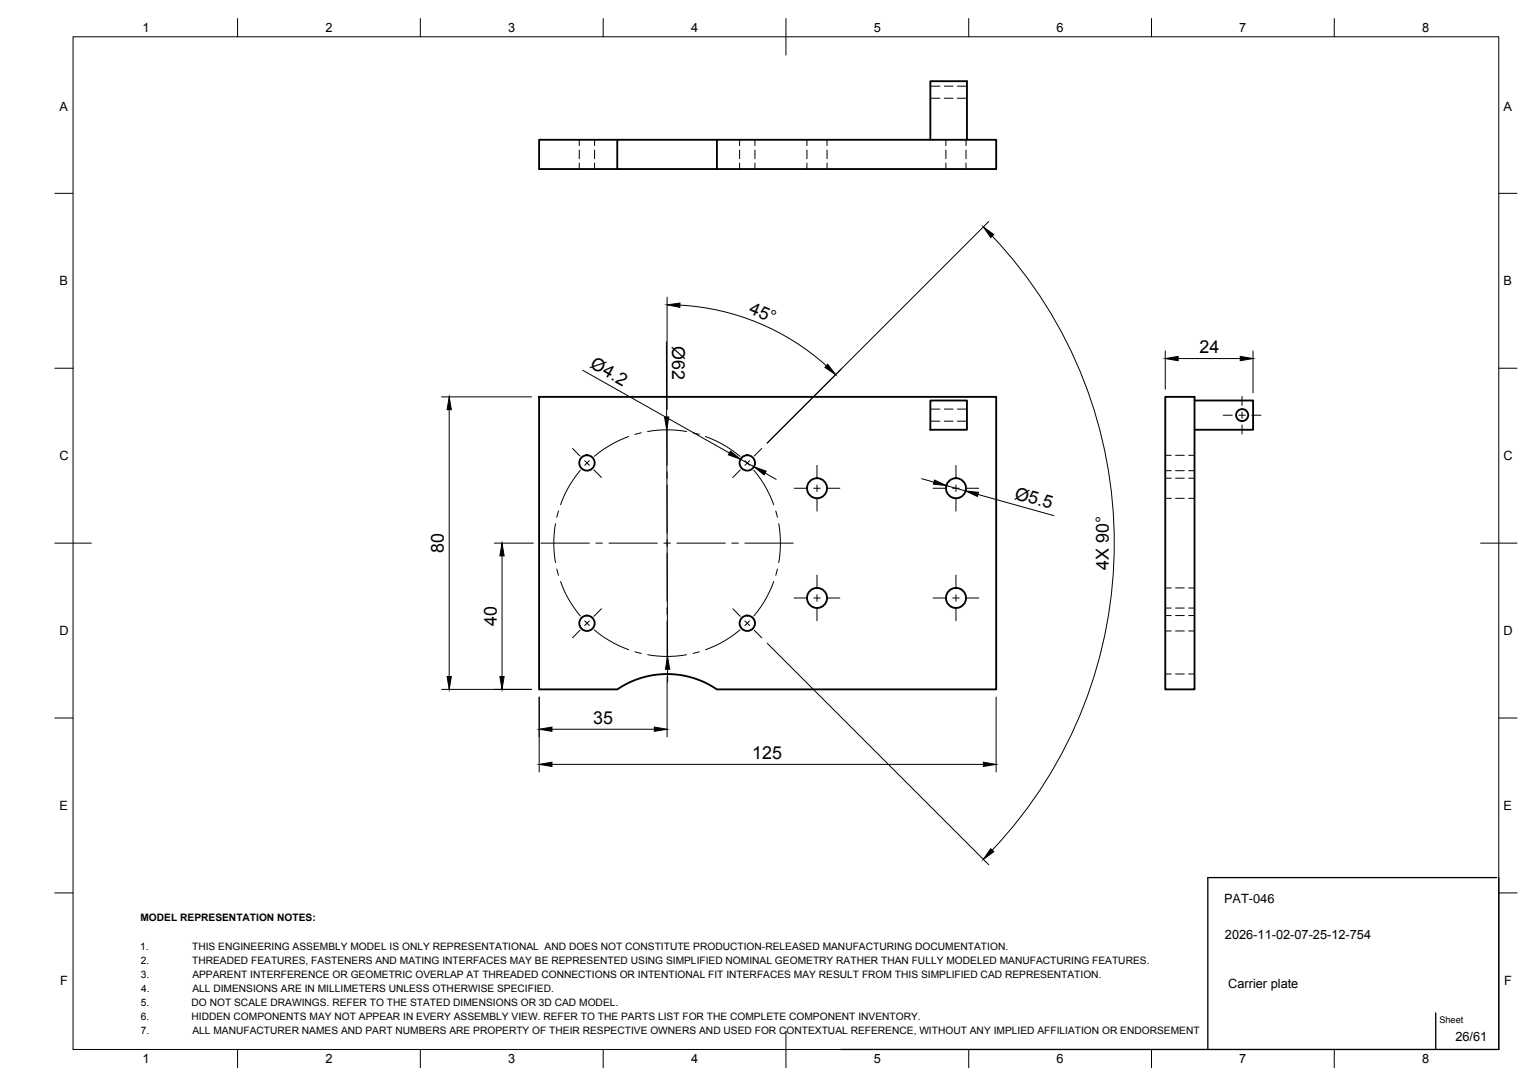
ISO-10303-21;
HEADER;
/* Generated by software containing ST-Developer
 * from STEP Tools, Inc. (www.steptools.com) 
 */

FILE_DESCRIPTION(
/* description */ ('Gear mesh backlash fixture'),
/* implementation_level */ '2;1');

FILE_NAME(
/* name */ 'Carrier plate.step',
/* time_stamp */ '2026-10-28T03:26:00-07:00',
/* author */ (''),
/* organization */ (''),
/* preprocessor_version */ 'ST-DEVELOPER v20.2',
/* originating_system */ 'Autodesk Translation Framework v15.17.0.0',
/* authorisation */ '');

FILE_SCHEMA (('AUTOMOTIVE_DESIGN { 1 0 10303 214 3 1 1 }'));
ENDSEC;

DATA;
#10=MECHANICAL_DESIGN_GEOMETRIC_PRESENTATION_REPRESENTATION('',(#1041),#57900);
#934=SHAPE_REPRESENTATION_RELATIONSHIP('SRR','None',#58131,#984);
#984=ADVANCED_BREP_SHAPE_REPRESENTATION('',(#1105),#57864);
#1041=STYLED_ITEM('',(#58451),#1105);
#1105=MANIFOLD_SOLID_BREP('Body1',#13602);
#1227=FACE_BOUND('',#2760,.T.);
#1228=FACE_BOUND('',#2763,.T.);
#1229=FACE_BOUND('',#2772,.T.);
#1230=FACE_BOUND('',#2773,.T.);
#1231=FACE_BOUND('',#2774,.T.);
#1232=FACE_BOUND('',#2775,.T.);
#1233=FACE_BOUND('',#2776,.T.);
#1234=FACE_BOUND('',#2777,.T.);
#1235=FACE_BOUND('',#2778,.T.);
#1236=FACE_BOUND('',#2779,.T.);
#1237=FACE_BOUND('',#2786,.T.);
#1238=FACE_BOUND('',#2787,.T.);
#1239=FACE_BOUND('',#2788,.T.);
#1240=FACE_BOUND('',#2789,.T.);
#1241=FACE_BOUND('',#2790,.T.);
#1242=FACE_BOUND('',#2791,.T.);
#1243=FACE_BOUND('',#2792,.T.);
#1244=FACE_BOUND('',#2793,.T.);
#1245=FACE_BOUND('',#2794,.T.);
#1440=PLANE('',#14667);
#1441=PLANE('',#14668);
#1442=PLANE('',#14669);
#1443=PLANE('',#14670);
#1444=PLANE('',#14671);
#1445=PLANE('',#14687);
#1446=PLANE('',#14688);
#1447=PLANE('',#14689);
#1448=PLANE('',#14690);
#1449=PLANE('',#14691);
#1450=PLANE('',#14692);
#1451=PLANE('',#14693);
#1905=FACE_OUTER_BOUND('',#2754,.T.);
#1906=FACE_OUTER_BOUND('',#2755,.T.);
#1907=FACE_OUTER_BOUND('',#2756,.T.);
#1908=FACE_OUTER_BOUND('',#2757,.T.);
#1909=FACE_OUTER_BOUND('',#2758,.T.);
#1910=FACE_OUTER_BOUND('',#2759,.T.);
#1911=FACE_OUTER_BOUND('',#2761,.T.);
#1912=FACE_OUTER_BOUND('',#2762,.T.);
#1913=FACE_OUTER_BOUND('',#2764,.T.);
#1914=FACE_OUTER_BOUND('',#2765,.T.);
#1915=FACE_OUTER_BOUND('',#2766,.T.);
#1916=FACE_OUTER_BOUND('',#2767,.T.);
#1917=FACE_OUTER_BOUND('',#2768,.T.);
#1918=FACE_OUTER_BOUND('',#2769,.T.);
#1919=FACE_OUTER_BOUND('',#2770,.T.);
#1920=FACE_OUTER_BOUND('',#2771,.T.);
#1921=FACE_OUTER_BOUND('',#2780,.T.);
#1922=FACE_OUTER_BOUND('',#2781,.T.);
#1923=FACE_OUTER_BOUND('',#2782,.T.);
#1924=FACE_OUTER_BOUND('',#2783,.T.);
#1925=FACE_OUTER_BOUND('',#2784,.T.);
#1926=FACE_OUTER_BOUND('',#2785,.T.);
#2754=EDGE_LOOP('',(#9809,#9810,#9811,#9812));
#2755=EDGE_LOOP('',(#9813,#9814,#9815,#9816));
#2756=EDGE_LOOP('',(#9817,#9818,#9819,#9820));
#2757=EDGE_LOOP('',(#9821,#9822,#9823,#9824));
#2758=EDGE_LOOP('',(#9825,#9826,#9827,#9828));
#2759=EDGE_LOOP('',(#9829,#9830,#9831,#9832));
#2760=EDGE_LOOP('',(#9833));
#2761=EDGE_LOOP('',(#9834,#9835,#9836,#9837));
#2762=EDGE_LOOP('',(#9838,#9839,#9840,#9841));
#2763=EDGE_LOOP('',(#9842));
#2764=EDGE_LOOP('',(#9843,#9844,#9845,#9846));
#2765=EDGE_LOOP('',(#9847,#9848,#9849,#9850));
#2766=EDGE_LOOP('',(#9851,#9852,#9853,#9854));
#2767=EDGE_LOOP('',(#9855,#9856,#9857,#9858));
#2768=EDGE_LOOP('',(#9859,#9860,#9861,#9862));
#2769=EDGE_LOOP('',(#9863,#9864,#9865,#9866));
#2770=EDGE_LOOP('',(#9867,#9868,#9869,#9870));
#2771=EDGE_LOOP('',(#9871,#9872,#9873,#9874,#9875,#9876));
#2772=EDGE_LOOP('',(#9877));
#2773=EDGE_LOOP('',(#9878));
#2774=EDGE_LOOP('',(#9879));
#2775=EDGE_LOOP('',(#9880));
#2776=EDGE_LOOP('',(#9881));
#2777=EDGE_LOOP('',(#9882));
#2778=EDGE_LOOP('',(#9883));
#2779=EDGE_LOOP('',(#9884));
#2780=EDGE_LOOP('',(#9885,#9886,#9887,#9888));
#2781=EDGE_LOOP('',(#9889,#9890,#9891,#9892));
#2782=EDGE_LOOP('',(#9893,#9894,#9895,#9896));
#2783=EDGE_LOOP('',(#9897,#9898,#9899,#9900));
#2784=EDGE_LOOP('',(#9901,#9902,#9903,#9904));
#2785=EDGE_LOOP('',(#9905,#9906,#9907,#9908,#9909,#9910));
#2786=EDGE_LOOP('',(#9911));
#2787=EDGE_LOOP('',(#9912));
#2788=EDGE_LOOP('',(#9913));
#2789=EDGE_LOOP('',(#9914));
#2790=EDGE_LOOP('',(#9915,#9916,#9917,#9918));
#2791=EDGE_LOOP('',(#9919));
#2792=EDGE_LOOP('',(#9920));
#2793=EDGE_LOOP('',(#9921));
#2794=EDGE_LOOP('',(#9922));
#3637=LINE('',#20642,#4526);
#3638=LINE('',#20648,#4527);
#3639=LINE('',#20654,#4528);
#3640=LINE('',#20660,#4529);
#3641=LINE('',#20666,#4530);
#3642=LINE('',#20671,#4531);
#3643=LINE('',#20673,#4532);
#3644=LINE('',#20675,#4533);
#3645=LINE('',#20676,#4534);
#3646=LINE('',#20679,#4535);
#3647=LINE('',#20681,#4536);
#3648=LINE('',#20682,#4537);
#3649=LINE('',#20685,#4538);
#3650=LINE('',#20687,#4539);
#3651=LINE('',#20688,#4540);
#3652=LINE('',#20690,#4541);
#3653=LINE('',#20691,#4542);
#3654=LINE('',#20697,#4543);
#3655=LINE('',#20703,#4544);
#3656=LINE('',#20709,#4545);
#3657=LINE('',#20715,#4546);
#3658=LINE('',#20720,#4547);
#3659=LINE('',#20724,#4548);
#3660=LINE('',#20728,#4549);
#3661=LINE('',#20730,#4550);
#3662=LINE('',#20732,#4551);
#3663=LINE('',#20734,#4552);
#3664=LINE('',#20735,#4553);
#3665=LINE('',#20738,#4554);
#3666=LINE('',#20739,#4555);
#3667=LINE('',#20742,#4556);
#3668=LINE('',#20743,#4557);
#3669=LINE('',#20746,#4558);
#3670=LINE('',#20747,#4559);
#3671=LINE('',#20750,#4560);
#3672=LINE('',#20751,#4561);
#3673=LINE('',#20753,#4562);
#4526=VECTOR('',#16722,0.21);
#4527=VECTOR('',#16729,0.21);
#4528=VECTOR('',#16736,0.210000000000001);
#4529=VECTOR('',#16743,0.210000000000001);
#4530=VECTOR('',#16750,0.164999999999999);
#4531=VECTOR('',#16755,1.);
#4532=VECTOR('',#16756,1.);
#4533=VECTOR('',#16757,1.);
#4534=VECTOR('',#16758,1.);
#4535=VECTOR('',#16761,1.);
#4536=VECTOR('',#16762,1.);
#4537=VECTOR('',#16763,1.);
#4538=VECTOR('',#16766,1.);
#4539=VECTOR('',#16767,1.);
#4540=VECTOR('',#16768,1.);
#4541=VECTOR('',#16771,1.);
#4542=VECTOR('',#16772,1.);
#4543=VECTOR('',#16779,0.275);
#4544=VECTOR('',#16786,0.275);
#4545=VECTOR('',#16793,0.275);
#4546=VECTOR('',#16800,0.275);
#4547=VECTOR('',#16805,1.);
#4548=VECTOR('',#16808,1.);
#4549=VECTOR('',#16813,1.);
#4550=VECTOR('',#16814,1.);
#4551=VECTOR('',#16815,1.);
#4552=VECTOR('',#16816,1.);
#4553=VECTOR('',#16817,1.);
#4554=VECTOR('',#16820,1.);
#4555=VECTOR('',#16821,1.);
#4556=VECTOR('',#16824,1.);
#4557=VECTOR('',#16825,1.);
#4558=VECTOR('',#16828,1.);
#4559=VECTOR('',#16829,1.);
#4560=VECTOR('',#16832,1.);
#4561=VECTOR('',#16833,1.);
#4562=VECTOR('',#16836,1.);
#5407=CIRCLE('',#14653,0.21);
#5408=CIRCLE('',#14654,0.21);
#5409=CIRCLE('',#14656,0.21);
#5410=CIRCLE('',#14657,0.21);
#5411=CIRCLE('',#14659,0.210000000000001);
#5412=CIRCLE('',#14660,0.210000000000001);
#5413=CIRCLE('',#14662,0.210000000000001);
#5414=CIRCLE('',#14663,0.210000000000001);
#5415=CIRCLE('',#14665,0.164999999999999);
#5416=CIRCLE('',#14666,0.164999999999999);
#5417=CIRCLE('',#14673,0.275);
#5418=CIRCLE('',#14674,0.275);
#5419=CIRCLE('',#14676,0.275);
#5420=CIRCLE('',#14677,0.275);
#5421=CIRCLE('',#14679,0.275);
#5422=CIRCLE('',#14680,0.275);
#5423=CIRCLE('',#14682,0.275);
#5424=CIRCLE('',#14683,0.275);
#5425=CIRCLE('',#14685,2.42);
#5426=CIRCLE('',#14686,2.42);
#6093=VERTEX_POINT('',#20639);
#6094=VERTEX_POINT('',#20641);
#6095=VERTEX_POINT('',#20645);
#6096=VERTEX_POINT('',#20647);
#6097=VERTEX_POINT('',#20651);
#6098=VERTEX_POINT('',#20653);
#6099=VERTEX_POINT('',#20657);
#6100=VERTEX_POINT('',#20659);
#6101=VERTEX_POINT('',#20663);
#6102=VERTEX_POINT('',#20665);
#6103=VERTEX_POINT('',#20669);
#6104=VERTEX_POINT('',#20670);
#6105=VERTEX_POINT('',#20672);
#6106=VERTEX_POINT('',#20674);
#6107=VERTEX_POINT('',#20678);
#6108=VERTEX_POINT('',#20680);
#6109=VERTEX_POINT('',#20684);
#6110=VERTEX_POINT('',#20686);
#6111=VERTEX_POINT('',#20694);
#6112=VERTEX_POINT('',#20696);
#6113=VERTEX_POINT('',#20700);
#6114=VERTEX_POINT('',#20702);
#6115=VERTEX_POINT('',#20706);
#6116=VERTEX_POINT('',#20708);
#6117=VERTEX_POINT('',#20712);
#6118=VERTEX_POINT('',#20714);
#6119=VERTEX_POINT('',#20718);
#6120=VERTEX_POINT('',#20719);
#6121=VERTEX_POINT('',#20721);
#6122=VERTEX_POINT('',#20723);
#6123=VERTEX_POINT('',#20727);
#6124=VERTEX_POINT('',#20729);
#6125=VERTEX_POINT('',#20731);
#6126=VERTEX_POINT('',#20733);
#6127=VERTEX_POINT('',#20737);
#6128=VERTEX_POINT('',#20741);
#6129=VERTEX_POINT('',#20745);
#6130=VERTEX_POINT('',#20749);
#7491=EDGE_CURVE('',#6093,#6093,#5407,.T.);
#7492=EDGE_CURVE('',#6093,#6094,#3637,.T.);
#7493=EDGE_CURVE('',#6094,#6094,#5408,.T.);
#7494=EDGE_CURVE('',#6095,#6095,#5409,.T.);
#7495=EDGE_CURVE('',#6095,#6096,#3638,.T.);
#7496=EDGE_CURVE('',#6096,#6096,#5410,.T.);
#7497=EDGE_CURVE('',#6097,#6097,#5411,.T.);
#7498=EDGE_CURVE('',#6097,#6098,#3639,.T.);
#7499=EDGE_CURVE('',#6098,#6098,#5412,.T.);
#7500=EDGE_CURVE('',#6099,#6099,#5413,.T.);
#7501=EDGE_CURVE('',#6099,#6100,#3640,.T.);
#7502=EDGE_CURVE('',#6100,#6100,#5414,.T.);
#7503=EDGE_CURVE('',#6101,#6101,#5415,.T.);
#7504=EDGE_CURVE('',#6101,#6102,#3641,.T.);
#7505=EDGE_CURVE('',#6102,#6102,#5416,.T.);
#7506=EDGE_CURVE('',#6103,#6104,#3642,.T.);
#7507=EDGE_CURVE('',#6104,#6105,#3643,.T.);
#7508=EDGE_CURVE('',#6106,#6105,#3644,.T.);
#7509=EDGE_CURVE('',#6103,#6106,#3645,.T.);
#7510=EDGE_CURVE('',#6107,#6103,#3646,.T.);
#7511=EDGE_CURVE('',#6108,#6106,#3647,.T.);
#7512=EDGE_CURVE('',#6107,#6108,#3648,.T.);
#7513=EDGE_CURVE('',#6109,#6107,#3649,.T.);
#7514=EDGE_CURVE('',#6110,#6108,#3650,.T.);
#7515=EDGE_CURVE('',#6109,#6110,#3651,.T.);
#7516=EDGE_CURVE('',#6104,#6109,#3652,.T.);
#7517=EDGE_CURVE('',#6105,#6110,#3653,.T.);
#7518=EDGE_CURVE('',#6111,#6111,#5417,.T.);
#7519=EDGE_CURVE('',#6111,#6112,#3654,.T.);
#7520=EDGE_CURVE('',#6112,#6112,#5418,.T.);
#7521=EDGE_CURVE('',#6113,#6113,#5419,.T.);
#7522=EDGE_CURVE('',#6113,#6114,#3655,.T.);
#7523=EDGE_CURVE('',#6114,#6114,#5420,.T.);
#7524=EDGE_CURVE('',#6115,#6115,#5421,.T.);
#7525=EDGE_CURVE('',#6115,#6116,#3656,.T.);
#7526=EDGE_CURVE('',#6116,#6116,#5422,.T.);
#7527=EDGE_CURVE('',#6117,#6117,#5423,.T.);
#7528=EDGE_CURVE('',#6117,#6118,#3657,.T.);
#7529=EDGE_CURVE('',#6118,#6118,#5424,.T.);
#7530=EDGE_CURVE('',#6119,#6120,#3658,.T.);
#7531=EDGE_CURVE('',#6121,#6119,#5425,.T.);
#7532=EDGE_CURVE('',#6122,#6121,#3659,.T.);
#7533=EDGE_CURVE('',#6120,#6122,#5426,.T.);
#7534=EDGE_CURVE('',#6119,#6123,#3660,.T.);
#7535=EDGE_CURVE('',#6123,#6124,#3661,.T.);
#7536=EDGE_CURVE('',#6124,#6125,#3662,.T.);
#7537=EDGE_CURVE('',#6125,#6126,#3663,.T.);
#7538=EDGE_CURVE('',#6126,#6121,#3664,.T.);
#7539=EDGE_CURVE('',#6120,#6127,#3665,.T.);
#7540=EDGE_CURVE('',#6127,#6123,#3666,.T.);
#7541=EDGE_CURVE('',#6128,#6126,#3667,.T.);
#7542=EDGE_CURVE('',#6128,#6122,#3668,.T.);
#7543=EDGE_CURVE('',#6129,#6128,#3669,.T.);
#7544=EDGE_CURVE('',#6129,#6125,#3670,.T.);
#7545=EDGE_CURVE('',#6130,#6129,#3671,.T.);
#7546=EDGE_CURVE('',#6130,#6124,#3672,.T.);
#7547=EDGE_CURVE('',#6127,#6130,#3673,.T.);
#9809=ORIENTED_EDGE('',*,*,#7491,.F.);
#9810=ORIENTED_EDGE('',*,*,#7492,.T.);
#9811=ORIENTED_EDGE('',*,*,#7493,.F.);
#9812=ORIENTED_EDGE('',*,*,#7492,.F.);
#9813=ORIENTED_EDGE('',*,*,#7494,.F.);
#9814=ORIENTED_EDGE('',*,*,#7495,.T.);
#9815=ORIENTED_EDGE('',*,*,#7496,.F.);
#9816=ORIENTED_EDGE('',*,*,#7495,.F.);
#9817=ORIENTED_EDGE('',*,*,#7497,.F.);
#9818=ORIENTED_EDGE('',*,*,#7498,.T.);
#9819=ORIENTED_EDGE('',*,*,#7499,.F.);
#9820=ORIENTED_EDGE('',*,*,#7498,.F.);
#9821=ORIENTED_EDGE('',*,*,#7500,.F.);
#9822=ORIENTED_EDGE('',*,*,#7501,.T.);
#9823=ORIENTED_EDGE('',*,*,#7502,.F.);
#9824=ORIENTED_EDGE('',*,*,#7501,.F.);
#9825=ORIENTED_EDGE('',*,*,#7503,.F.);
#9826=ORIENTED_EDGE('',*,*,#7504,.T.);
#9827=ORIENTED_EDGE('',*,*,#7505,.F.);
#9828=ORIENTED_EDGE('',*,*,#7504,.F.);
#9829=ORIENTED_EDGE('',*,*,#7506,.T.);
#9830=ORIENTED_EDGE('',*,*,#7507,.T.);
#9831=ORIENTED_EDGE('',*,*,#7508,.F.);
#9832=ORIENTED_EDGE('',*,*,#7509,.F.);
#9833=ORIENTED_EDGE('',*,*,#7505,.T.);
#9834=ORIENTED_EDGE('',*,*,#7510,.T.);
#9835=ORIENTED_EDGE('',*,*,#7509,.T.);
#9836=ORIENTED_EDGE('',*,*,#7511,.F.);
#9837=ORIENTED_EDGE('',*,*,#7512,.F.);
#9838=ORIENTED_EDGE('',*,*,#7513,.T.);
#9839=ORIENTED_EDGE('',*,*,#7512,.T.);
#9840=ORIENTED_EDGE('',*,*,#7514,.F.);
#9841=ORIENTED_EDGE('',*,*,#7515,.F.);
#9842=ORIENTED_EDGE('',*,*,#7503,.T.);
#9843=ORIENTED_EDGE('',*,*,#7516,.T.);
#9844=ORIENTED_EDGE('',*,*,#7515,.T.);
#9845=ORIENTED_EDGE('',*,*,#7517,.F.);
#9846=ORIENTED_EDGE('',*,*,#7507,.F.);
#9847=ORIENTED_EDGE('',*,*,#7516,.F.);
#9848=ORIENTED_EDGE('',*,*,#7506,.F.);
#9849=ORIENTED_EDGE('',*,*,#7510,.F.);
#9850=ORIENTED_EDGE('',*,*,#7513,.F.);
#9851=ORIENTED_EDGE('',*,*,#7518,.F.);
#9852=ORIENTED_EDGE('',*,*,#7519,.T.);
#9853=ORIENTED_EDGE('',*,*,#7520,.F.);
#9854=ORIENTED_EDGE('',*,*,#7519,.F.);
#9855=ORIENTED_EDGE('',*,*,#7521,.F.);
#9856=ORIENTED_EDGE('',*,*,#7522,.T.);
#9857=ORIENTED_EDGE('',*,*,#7523,.F.);
#9858=ORIENTED_EDGE('',*,*,#7522,.F.);
#9859=ORIENTED_EDGE('',*,*,#7524,.F.);
#9860=ORIENTED_EDGE('',*,*,#7525,.T.);
#9861=ORIENTED_EDGE('',*,*,#7526,.F.);
#9862=ORIENTED_EDGE('',*,*,#7525,.F.);
#9863=ORIENTED_EDGE('',*,*,#7527,.F.);
#9864=ORIENTED_EDGE('',*,*,#7528,.T.);
#9865=ORIENTED_EDGE('',*,*,#7529,.F.);
#9866=ORIENTED_EDGE('',*,*,#7528,.F.);
#9867=ORIENTED_EDGE('',*,*,#7530,.F.);
#9868=ORIENTED_EDGE('',*,*,#7531,.F.);
#9869=ORIENTED_EDGE('',*,*,#7532,.F.);
#9870=ORIENTED_EDGE('',*,*,#7533,.F.);
#9871=ORIENTED_EDGE('',*,*,#7531,.T.);
#9872=ORIENTED_EDGE('',*,*,#7534,.T.);
#9873=ORIENTED_EDGE('',*,*,#7535,.T.);
#9874=ORIENTED_EDGE('',*,*,#7536,.T.);
#9875=ORIENTED_EDGE('',*,*,#7537,.T.);
#9876=ORIENTED_EDGE('',*,*,#7538,.T.);
#9877=ORIENTED_EDGE('',*,*,#7529,.T.);
#9878=ORIENTED_EDGE('',*,*,#7526,.T.);
#9879=ORIENTED_EDGE('',*,*,#7523,.T.);
#9880=ORIENTED_EDGE('',*,*,#7520,.T.);
#9881=ORIENTED_EDGE('',*,*,#7502,.T.);
#9882=ORIENTED_EDGE('',*,*,#7499,.T.);
#9883=ORIENTED_EDGE('',*,*,#7496,.T.);
#9884=ORIENTED_EDGE('',*,*,#7493,.T.);
#9885=ORIENTED_EDGE('',*,*,#7530,.T.);
#9886=ORIENTED_EDGE('',*,*,#7539,.T.);
#9887=ORIENTED_EDGE('',*,*,#7540,.T.);
#9888=ORIENTED_EDGE('',*,*,#7534,.F.);
#9889=ORIENTED_EDGE('',*,*,#7532,.T.);
#9890=ORIENTED_EDGE('',*,*,#7538,.F.);
#9891=ORIENTED_EDGE('',*,*,#7541,.F.);
#9892=ORIENTED_EDGE('',*,*,#7542,.T.);
#9893=ORIENTED_EDGE('',*,*,#7543,.T.);
#9894=ORIENTED_EDGE('',*,*,#7541,.T.);
#9895=ORIENTED_EDGE('',*,*,#7537,.F.);
#9896=ORIENTED_EDGE('',*,*,#7544,.F.);
#9897=ORIENTED_EDGE('',*,*,#7545,.T.);
#9898=ORIENTED_EDGE('',*,*,#7544,.T.);
#9899=ORIENTED_EDGE('',*,*,#7536,.F.);
#9900=ORIENTED_EDGE('',*,*,#7546,.F.);
#9901=ORIENTED_EDGE('',*,*,#7547,.T.);
#9902=ORIENTED_EDGE('',*,*,#7546,.T.);
#9903=ORIENTED_EDGE('',*,*,#7535,.F.);
#9904=ORIENTED_EDGE('',*,*,#7540,.F.);
#9905=ORIENTED_EDGE('',*,*,#7533,.T.);
#9906=ORIENTED_EDGE('',*,*,#7542,.F.);
#9907=ORIENTED_EDGE('',*,*,#7543,.F.);
#9908=ORIENTED_EDGE('',*,*,#7545,.F.);
#9909=ORIENTED_EDGE('',*,*,#7547,.F.);
#9910=ORIENTED_EDGE('',*,*,#7539,.F.);
#9911=ORIENTED_EDGE('',*,*,#7527,.T.);
#9912=ORIENTED_EDGE('',*,*,#7524,.T.);
#9913=ORIENTED_EDGE('',*,*,#7521,.T.);
#9914=ORIENTED_EDGE('',*,*,#7518,.T.);
#9915=ORIENTED_EDGE('',*,*,#7508,.T.);
#9916=ORIENTED_EDGE('',*,*,#7517,.T.);
#9917=ORIENTED_EDGE('',*,*,#7514,.T.);
#9918=ORIENTED_EDGE('',*,*,#7511,.T.);
#9919=ORIENTED_EDGE('',*,*,#7500,.T.);
#9920=ORIENTED_EDGE('',*,*,#7497,.T.);
#9921=ORIENTED_EDGE('',*,*,#7494,.T.);
#9922=ORIENTED_EDGE('',*,*,#7491,.T.);
#12662=CYLINDRICAL_SURFACE('',#14652,0.21);
#12663=CYLINDRICAL_SURFACE('',#14655,0.21);
#12664=CYLINDRICAL_SURFACE('',#14658,0.210000000000001);
#12665=CYLINDRICAL_SURFACE('',#14661,0.210000000000001);
#12666=CYLINDRICAL_SURFACE('',#14664,0.164999999999999);
#12667=CYLINDRICAL_SURFACE('',#14672,0.275);
#12668=CYLINDRICAL_SURFACE('',#14675,0.275);
#12669=CYLINDRICAL_SURFACE('',#14678,0.275);
#12670=CYLINDRICAL_SURFACE('',#14681,0.275);
#12671=CYLINDRICAL_SURFACE('',#14684,2.42);
#13022=ADVANCED_FACE('',(#1905),#12662,.F.);
#13023=ADVANCED_FACE('',(#1906),#12663,.F.);
#13024=ADVANCED_FACE('',(#1907),#12664,.F.);
#13025=ADVANCED_FACE('',(#1908),#12665,.F.);
#13026=ADVANCED_FACE('',(#1909),#12666,.F.);
#13027=ADVANCED_FACE('',(#1910,#1227),#1440,.T.);
#13028=ADVANCED_FACE('',(#1911),#1441,.T.);
#13029=ADVANCED_FACE('',(#1912,#1228),#1442,.T.);
#13030=ADVANCED_FACE('',(#1913),#1443,.T.);
#13031=ADVANCED_FACE('',(#1914),#1444,.F.);
#13032=ADVANCED_FACE('',(#1915),#12667,.F.);
#13033=ADVANCED_FACE('',(#1916),#12668,.F.);
#13034=ADVANCED_FACE('',(#1917),#12669,.F.);
#13035=ADVANCED_FACE('',(#1918),#12670,.F.);
#13036=ADVANCED_FACE('',(#1919),#12671,.F.);
#13037=ADVANCED_FACE('',(#1920,#1229,#1230,#1231,#1232,#1233,#1234,#1235,
#1236),#1445,.T.);
#13038=ADVANCED_FACE('',(#1921),#1446,.T.);
#13039=ADVANCED_FACE('',(#1922),#1447,.T.);
#13040=ADVANCED_FACE('',(#1923),#1448,.T.);
#13041=ADVANCED_FACE('',(#1924),#1449,.T.);
#13042=ADVANCED_FACE('',(#1925),#1450,.T.);
#13043=ADVANCED_FACE('',(#1926,#1237,#1238,#1239,#1240,#1241,#1242,#1243,
#1244,#1245),#1451,.F.);
#13602=CLOSED_SHELL('',(#13022,#13023,#13024,#13025,#13026,#13027,#13028,
#13029,#13030,#13031,#13032,#13033,#13034,#13035,#13036,#13037,#13038,#13039,
#13040,#13041,#13042,#13043));
#14651=AXIS2_PLACEMENT_3D('',#20637,#16716,#16717);
#14652=AXIS2_PLACEMENT_3D('',#20638,#16718,#16719);
#14653=AXIS2_PLACEMENT_3D('',#20640,#16720,#16721);
#14654=AXIS2_PLACEMENT_3D('',#20643,#16723,#16724);
#14655=AXIS2_PLACEMENT_3D('',#20644,#16725,#16726);
#14656=AXIS2_PLACEMENT_3D('',#20646,#16727,#16728);
#14657=AXIS2_PLACEMENT_3D('',#20649,#16730,#16731);
#14658=AXIS2_PLACEMENT_3D('',#20650,#16732,#16733);
#14659=AXIS2_PLACEMENT_3D('',#20652,#16734,#16735);
#14660=AXIS2_PLACEMENT_3D('',#20655,#16737,#16738);
#14661=AXIS2_PLACEMENT_3D('',#20656,#16739,#16740);
#14662=AXIS2_PLACEMENT_3D('',#20658,#16741,#16742);
#14663=AXIS2_PLACEMENT_3D('',#20661,#16744,#16745);
#14664=AXIS2_PLACEMENT_3D('',#20662,#16746,#16747);
#14665=AXIS2_PLACEMENT_3D('',#20664,#16748,#16749);
#14666=AXIS2_PLACEMENT_3D('',#20667,#16751,#16752);
#14667=AXIS2_PLACEMENT_3D('',#20668,#16753,#16754);
#14668=AXIS2_PLACEMENT_3D('',#20677,#16759,#16760);
#14669=AXIS2_PLACEMENT_3D('',#20683,#16764,#16765);
#14670=AXIS2_PLACEMENT_3D('',#20689,#16769,#16770);
#14671=AXIS2_PLACEMENT_3D('',#20692,#16773,#16774);
#14672=AXIS2_PLACEMENT_3D('',#20693,#16775,#16776);
#14673=AXIS2_PLACEMENT_3D('',#20695,#16777,#16778);
#14674=AXIS2_PLACEMENT_3D('',#20698,#16780,#16781);
#14675=AXIS2_PLACEMENT_3D('',#20699,#16782,#16783);
#14676=AXIS2_PLACEMENT_3D('',#20701,#16784,#16785);
#14677=AXIS2_PLACEMENT_3D('',#20704,#16787,#16788);
#14678=AXIS2_PLACEMENT_3D('',#20705,#16789,#16790);
#14679=AXIS2_PLACEMENT_3D('',#20707,#16791,#16792);
#14680=AXIS2_PLACEMENT_3D('',#20710,#16794,#16795);
#14681=AXIS2_PLACEMENT_3D('',#20711,#16796,#16797);
#14682=AXIS2_PLACEMENT_3D('',#20713,#16798,#16799);
#14683=AXIS2_PLACEMENT_3D('',#20716,#16801,#16802);
#14684=AXIS2_PLACEMENT_3D('',#20717,#16803,#16804);
#14685=AXIS2_PLACEMENT_3D('',#20722,#16806,#16807);
#14686=AXIS2_PLACEMENT_3D('',#20725,#16809,#16810);
#14687=AXIS2_PLACEMENT_3D('',#20726,#16811,#16812);
#14688=AXIS2_PLACEMENT_3D('',#20736,#16818,#16819);
#14689=AXIS2_PLACEMENT_3D('',#20740,#16822,#16823);
#14690=AXIS2_PLACEMENT_3D('',#20744,#16826,#16827);
#14691=AXIS2_PLACEMENT_3D('',#20748,#16830,#16831);
#14692=AXIS2_PLACEMENT_3D('',#20752,#16834,#16835);
#14693=AXIS2_PLACEMENT_3D('',#20754,#16837,#16838);
#16716=DIRECTION('axis',(0.,0.,1.));
#16717=DIRECTION('refdir',(1.,0.,0.));
#16718=DIRECTION('center_axis',(0.,0.,1.));
#16719=DIRECTION('ref_axis',(1.,0.,0.));
#16720=DIRECTION('center_axis',(0.,0.,1.));
#16721=DIRECTION('ref_axis',(1.,0.,0.));
#16722=DIRECTION('',(0.,0.,1.));
#16723=DIRECTION('center_axis',(0.,0.,-1.));
#16724=DIRECTION('ref_axis',(1.,0.,0.));
#16725=DIRECTION('center_axis',(0.,0.,1.));
#16726=DIRECTION('ref_axis',(1.,0.,0.));
#16727=DIRECTION('center_axis',(0.,0.,1.));
#16728=DIRECTION('ref_axis',(1.,0.,0.));
#16729=DIRECTION('',(0.,0.,1.));
#16730=DIRECTION('center_axis',(0.,0.,-1.));
#16731=DIRECTION('ref_axis',(1.,0.,0.));
#16732=DIRECTION('center_axis',(0.,0.,1.));
#16733=DIRECTION('ref_axis',(1.,0.,0.));
#16734=DIRECTION('center_axis',(0.,0.,1.));
#16735=DIRECTION('ref_axis',(1.,0.,0.));
#16736=DIRECTION('',(0.,0.,1.));
#16737=DIRECTION('center_axis',(0.,0.,-1.));
#16738=DIRECTION('ref_axis',(1.,0.,0.));
#16739=DIRECTION('center_axis',(0.,0.,1.));
#16740=DIRECTION('ref_axis',(1.,0.,0.));
#16741=DIRECTION('center_axis',(0.,0.,1.));
#16742=DIRECTION('ref_axis',(1.,0.,0.));
#16743=DIRECTION('',(0.,0.,1.));
#16744=DIRECTION('center_axis',(0.,0.,-1.));
#16745=DIRECTION('ref_axis',(1.,0.,0.));
#16746=DIRECTION('center_axis',(0.,1.,0.));
#16747=DIRECTION('ref_axis',(1.,0.,0.));
#16748=DIRECTION('center_axis',(0.,1.,0.));
#16749=DIRECTION('ref_axis',(1.,0.,0.));
#16750=DIRECTION('',(0.,1.,0.));
#16751=DIRECTION('center_axis',(0.,-1.,0.));
#16752=DIRECTION('ref_axis',(1.,0.,0.));
#16753=DIRECTION('center_axis',(0.,1.,0.));
#16754=DIRECTION('ref_axis',(-1.,0.,0.));
#16755=DIRECTION('',(-1.,0.,0.));
#16756=DIRECTION('',(0.,0.,1.));
#16757=DIRECTION('',(-1.,0.,0.));
#16758=DIRECTION('',(0.,0.,1.));
#16759=DIRECTION('center_axis',(1.,0.,0.));
#16760=DIRECTION('ref_axis',(0.,1.,0.));
#16761=DIRECTION('',(0.,1.,0.));
#16762=DIRECTION('',(0.,1.,0.));
#16763=DIRECTION('',(0.,0.,1.));
#16764=DIRECTION('center_axis',(0.,-1.,0.));
#16765=DIRECTION('ref_axis',(1.,0.,0.));
#16766=DIRECTION('',(1.,0.,0.));
#16767=DIRECTION('',(1.,0.,0.));
#16768=DIRECTION('',(0.,0.,1.));
#16769=DIRECTION('center_axis',(-1.,0.,0.));
#16770=DIRECTION('ref_axis',(0.,-1.,0.));
#16771=DIRECTION('',(0.,-1.,0.));
#16772=DIRECTION('',(0.,-1.,0.));
#16773=DIRECTION('center_axis',(0.,0.,1.));
#16774=DIRECTION('ref_axis',(1.,0.,0.));
#16775=DIRECTION('center_axis',(0.,0.,1.));
#16776=DIRECTION('ref_axis',(1.,0.,0.));
#16777=DIRECTION('center_axis',(0.,0.,1.));
#16778=DIRECTION('ref_axis',(1.,0.,0.));
#16779=DIRECTION('',(0.,0.,1.));
#16780=DIRECTION('center_axis',(0.,0.,-1.));
#16781=DIRECTION('ref_axis',(1.,0.,0.));
#16782=DIRECTION('center_axis',(0.,0.,1.));
#16783=DIRECTION('ref_axis',(1.,0.,0.));
#16784=DIRECTION('center_axis',(0.,0.,1.));
#16785=DIRECTION('ref_axis',(1.,0.,0.));
#16786=DIRECTION('',(0.,0.,1.));
#16787=DIRECTION('center_axis',(0.,0.,-1.));
#16788=DIRECTION('ref_axis',(1.,0.,0.));
#16789=DIRECTION('center_axis',(0.,0.,1.));
#16790=DIRECTION('ref_axis',(1.,0.,0.));
#16791=DIRECTION('center_axis',(0.,0.,1.));
#16792=DIRECTION('ref_axis',(1.,0.,0.));
#16793=DIRECTION('',(0.,0.,1.));
#16794=DIRECTION('center_axis',(0.,0.,-1.));
#16795=DIRECTION('ref_axis',(1.,0.,0.));
#16796=DIRECTION('center_axis',(0.,0.,1.));
#16797=DIRECTION('ref_axis',(1.,0.,0.));
#16798=DIRECTION('center_axis',(0.,0.,1.));
#16799=DIRECTION('ref_axis',(1.,0.,0.));
#16800=DIRECTION('',(0.,0.,1.));
#16801=DIRECTION('center_axis',(0.,0.,-1.));
#16802=DIRECTION('ref_axis',(1.,0.,0.));
#16803=DIRECTION('center_axis',(0.,0.,1.));
#16804=DIRECTION('ref_axis',(1.,0.,0.));
#16805=DIRECTION('',(0.,0.,-1.));
#16806=DIRECTION('center_axis',(0.,0.,-1.));
#16807=DIRECTION('ref_axis',(1.,0.,0.));
#16808=DIRECTION('',(0.,0.,1.));
#16809=DIRECTION('center_axis',(0.,0.,1.));
#16810=DIRECTION('ref_axis',(1.,0.,0.));
#16811=DIRECTION('center_axis',(0.,0.,1.));
#16812=DIRECTION('ref_axis',(1.,0.,0.));
#16813=DIRECTION('',(0.,-1.,0.));
#16814=DIRECTION('',(1.,0.,0.));
#16815=DIRECTION('',(0.,1.,0.));
#16816=DIRECTION('',(-1.,0.,0.));
#16817=DIRECTION('',(0.,-1.,0.));
#16818=DIRECTION('center_axis',(-1.,0.,0.));
#16819=DIRECTION('ref_axis',(0.,-1.,0.));
#16820=DIRECTION('',(0.,-1.,0.));
#16821=DIRECTION('',(0.,0.,1.));
#16822=DIRECTION('center_axis',(-1.,0.,0.));
#16823=DIRECTION('ref_axis',(0.,-1.,0.));
#16824=DIRECTION('',(0.,0.,1.));
#16825=DIRECTION('',(0.,-1.,0.));
#16826=DIRECTION('center_axis',(0.,1.,0.));
#16827=DIRECTION('ref_axis',(-1.,0.,0.));
#16828=DIRECTION('',(-1.,0.,0.));
#16829=DIRECTION('',(0.,0.,1.));
#16830=DIRECTION('center_axis',(1.,0.,0.));
#16831=DIRECTION('ref_axis',(0.,1.,0.));
#16832=DIRECTION('',(0.,1.,0.));
#16833=DIRECTION('',(0.,0.,1.));
#16834=DIRECTION('center_axis',(0.,-1.,0.));
#16835=DIRECTION('ref_axis',(1.,0.,0.));
#16836=DIRECTION('',(1.,0.,0.));
#16837=DIRECTION('center_axis',(0.,0.,1.));
#16838=DIRECTION('ref_axis',(1.,0.,0.));
#20637=CARTESIAN_POINT('',(0.,0.,0.));
#20638=CARTESIAN_POINT('Origin',(3.8079689783217,-2.1920310216783,2.3));
#20639=CARTESIAN_POINT('',(3.5979689783217,-2.1920310216783,2.4));
#20640=CARTESIAN_POINT('Origin',(3.8079689783217,-2.1920310216783,2.4));
#20641=CARTESIAN_POINT('',(3.5979689783217,-2.1920310216783,3.2));
#20642=CARTESIAN_POINT('',(3.5979689783217,-2.1920310216783,2.3));
#20643=CARTESIAN_POINT('Origin',(3.8079689783217,-2.1920310216783,3.2));
#20644=CARTESIAN_POINT('Origin',(3.8079689783217,2.1920310216783,2.3));
#20645=CARTESIAN_POINT('',(3.5979689783217,2.1920310216783,2.4));
#20646=CARTESIAN_POINT('Origin',(3.8079689783217,2.1920310216783,2.4));
#20647=CARTESIAN_POINT('',(3.5979689783217,2.1920310216783,3.2));
#20648=CARTESIAN_POINT('',(3.5979689783217,2.1920310216783,2.3));
#20649=CARTESIAN_POINT('Origin',(3.8079689783217,2.1920310216783,3.2));
#20650=CARTESIAN_POINT('Origin',(8.1920310216783,2.1920310216783,2.3));
#20651=CARTESIAN_POINT('',(7.9820310216783,2.1920310216783,2.4));
#20652=CARTESIAN_POINT('Origin',(8.1920310216783,2.1920310216783,2.4));
#20653=CARTESIAN_POINT('',(7.9820310216783,2.1920310216783,3.2));
#20654=CARTESIAN_POINT('',(7.9820310216783,2.1920310216783,2.3));
#20655=CARTESIAN_POINT('Origin',(8.1920310216783,2.1920310216783,3.2));
#20656=CARTESIAN_POINT('Origin',(8.1920310216783,-2.1920310216783,2.3));
#20657=CARTESIAN_POINT('',(7.9820310216783,-2.1920310216783,2.4));
#20658=CARTESIAN_POINT('Origin',(8.1920310216783,-2.1920310216783,2.4));
#20659=CARTESIAN_POINT('',(7.9820310216783,-2.1920310216783,3.2));
#20660=CARTESIAN_POINT('',(7.9820310216783,-2.1920310216783,2.3));
#20661=CARTESIAN_POINT('Origin',(8.1920310216783,-2.1920310216783,3.2));
#20662=CARTESIAN_POINT('Origin',(9.5,7.19,1.1));
#20663=CARTESIAN_POINT('',(9.335,7.2,1.1));
#20664=CARTESIAN_POINT('Origin',(9.5,7.2,1.1));
#20665=CARTESIAN_POINT('',(9.335,8.2,1.1));
#20666=CARTESIAN_POINT('',(9.335,7.19,1.1));
#20667=CARTESIAN_POINT('Origin',(9.5,8.2,1.1));
#20668=CARTESIAN_POINT('Origin',(9.9,8.2,0.8));
#20669=CARTESIAN_POINT('',(9.9,8.2,0.8));
#20670=CARTESIAN_POINT('',(9.1,8.2,0.8));
#20671=CARTESIAN_POINT('',(9.9,8.2,0.8));
#20672=CARTESIAN_POINT('',(9.1,8.2,2.4));
#20673=CARTESIAN_POINT('',(9.1,8.2,0.8));
#20674=CARTESIAN_POINT('',(9.9,8.2,2.4));
#20675=CARTESIAN_POINT('',(7.95,8.2,2.4));
#20676=CARTESIAN_POINT('',(9.9,8.2,0.8));
#20677=CARTESIAN_POINT('Origin',(9.9,7.2,0.8));
#20678=CARTESIAN_POINT('',(9.9,7.2,0.8));
#20679=CARTESIAN_POINT('',(9.9,7.2,0.8));
#20680=CARTESIAN_POINT('',(9.9,7.2,2.4));
#20681=CARTESIAN_POINT('',(9.9,4.975,2.4));
#20682=CARTESIAN_POINT('',(9.9,7.2,0.8));
#20683=CARTESIAN_POINT('Origin',(9.1,7.2,0.8));
#20684=CARTESIAN_POINT('',(9.1,7.2,0.8));
#20685=CARTESIAN_POINT('',(9.1,7.2,0.8));
#20686=CARTESIAN_POINT('',(9.1,7.2,2.4));
#20687=CARTESIAN_POINT('',(7.55,7.2,2.4));
#20688=CARTESIAN_POINT('',(9.1,7.2,0.8));
#20689=CARTESIAN_POINT('Origin',(9.1,8.2,0.8));
#20690=CARTESIAN_POINT('',(9.1,8.2,0.8));
#20691=CARTESIAN_POINT('',(9.1,5.475,2.4));
#20692=CARTESIAN_POINT('Origin',(9.5,7.7,0.8));
#20693=CARTESIAN_POINT('Origin',(7.5,4.1,2.3));
#20694=CARTESIAN_POINT('',(7.225,4.1,2.4));
#20695=CARTESIAN_POINT('Origin',(7.5,4.1,2.4));
#20696=CARTESIAN_POINT('',(7.225,4.1,3.2));
#20697=CARTESIAN_POINT('',(7.225,4.1,2.3));
#20698=CARTESIAN_POINT('Origin',(7.5,4.1,3.2));
#20699=CARTESIAN_POINT('Origin',(4.5,7.9,2.3));
#20700=CARTESIAN_POINT('',(4.225,7.9,2.4));
#20701=CARTESIAN_POINT('Origin',(4.5,7.9,2.4));
#20702=CARTESIAN_POINT('',(4.225,7.9,3.2));
#20703=CARTESIAN_POINT('',(4.225,7.9,2.3));
#20704=CARTESIAN_POINT('Origin',(4.5,7.9,3.2));
#20705=CARTESIAN_POINT('Origin',(4.5,4.1,2.3));
#20706=CARTESIAN_POINT('',(4.225,4.1,2.4));
#20707=CARTESIAN_POINT('Origin',(4.5,4.1,2.4));
#20708=CARTESIAN_POINT('',(4.225,4.1,3.2));
#20709=CARTESIAN_POINT('',(4.225,4.1,2.3));
#20710=CARTESIAN_POINT('Origin',(4.5,4.1,3.2));
#20711=CARTESIAN_POINT('Origin',(7.5,7.9,2.3));
#20712=CARTESIAN_POINT('',(7.225,7.9,2.4));
#20713=CARTESIAN_POINT('Origin',(7.5,7.9,2.4));
#20714=CARTESIAN_POINT('',(7.225,7.9,3.2));
#20715=CARTESIAN_POINT('',(7.225,7.9,2.3));
#20716=CARTESIAN_POINT('Origin',(7.5,7.9,3.2));
#20717=CARTESIAN_POINT('Origin',(0.,0.,2.3));
#20718=CARTESIAN_POINT('',(2.,-1.36249770642009,3.2));
#20719=CARTESIAN_POINT('',(2.,-1.36249770642009,2.4));
#20720=CARTESIAN_POINT('',(2.,-1.36249770642009,2.3));
#20721=CARTESIAN_POINT('',(2.,1.36249770642009,3.2));
#20722=CARTESIAN_POINT('Origin',(0.,0.,3.2));
#20723=CARTESIAN_POINT('',(2.,1.36249770642009,2.4));
#20724=CARTESIAN_POINT('',(2.,1.36249770642009,2.3));
#20725=CARTESIAN_POINT('Origin',(0.,0.,2.4));
#20726=CARTESIAN_POINT('Origin',(6.,2.75,3.2));
#20727=CARTESIAN_POINT('',(2.,-3.5,3.2));
#20728=CARTESIAN_POINT('',(2.,9.,3.2));
#20729=CARTESIAN_POINT('',(10.,-3.5,3.2));
#20730=CARTESIAN_POINT('',(2.,-3.5,3.2));
#20731=CARTESIAN_POINT('',(10.,9.,3.2));
#20732=CARTESIAN_POINT('',(10.,-3.5,3.2));
#20733=CARTESIAN_POINT('',(2.,9.,3.2));
#20734=CARTESIAN_POINT('',(10.,9.,3.2));
#20735=CARTESIAN_POINT('',(2.,9.,3.2));
#20736=CARTESIAN_POINT('Origin',(2.,9.,2.4));
#20737=CARTESIAN_POINT('',(2.,-3.5,2.4));
#20738=CARTESIAN_POINT('',(2.,9.,2.4));
#20739=CARTESIAN_POINT('',(2.,-3.5,2.4));
#20740=CARTESIAN_POINT('Origin',(2.,9.,2.4));
#20741=CARTESIAN_POINT('',(2.,9.,2.4));
#20742=CARTESIAN_POINT('',(2.,9.,2.4));
#20743=CARTESIAN_POINT('',(2.,9.,2.4));
#20744=CARTESIAN_POINT('Origin',(10.,9.,2.4));
#20745=CARTESIAN_POINT('',(10.,9.,2.4));
#20746=CARTESIAN_POINT('',(10.,9.,2.4));
#20747=CARTESIAN_POINT('',(10.,9.,2.4));
#20748=CARTESIAN_POINT('Origin',(10.,-3.5,2.4));
#20749=CARTESIAN_POINT('',(10.,-3.5,2.4));
#20750=CARTESIAN_POINT('',(10.,-3.5,2.4));
#20751=CARTESIAN_POINT('',(10.,-3.5,2.4));
#20752=CARTESIAN_POINT('Origin',(2.,-3.5,2.4));
#20753=CARTESIAN_POINT('',(2.,-3.5,2.4));
#20754=CARTESIAN_POINT('Origin',(6.,2.75,2.4));
#57805=UNCERTAINTY_MEASURE_WITH_UNIT(LENGTH_MEASURE(0.001),#57901,
'DISTANCE_ACCURACY_VALUE',
'Maximum model space distance between geometric entities at asserted c
onnectivities');
#57841=UNCERTAINTY_MEASURE_WITH_UNIT(LENGTH_MEASURE(0.001),#57901,
'DISTANCE_ACCURACY_VALUE',
'Maximum model space distance between geometric entities at asserted c
onnectivities');
#57864=(
GEOMETRIC_REPRESENTATION_CONTEXT(3)
GLOBAL_UNCERTAINTY_ASSIGNED_CONTEXT((#57805))
GLOBAL_UNIT_ASSIGNED_CONTEXT((#57901,#57903,#57904))
REPRESENTATION_CONTEXT('','3D')
);
#57900=(
GEOMETRIC_REPRESENTATION_CONTEXT(3)
GLOBAL_UNCERTAINTY_ASSIGNED_CONTEXT((#57841))
GLOBAL_UNIT_ASSIGNED_CONTEXT((#57901,#57903,#57904))
REPRESENTATION_CONTEXT('','3D')
);
#57901=(
LENGTH_UNIT()
NAMED_UNIT(*)
SI_UNIT(.CENTI.,.METRE.)
);
#57903=(
NAMED_UNIT(*)
PLANE_ANGLE_UNIT()
SI_UNIT($,.RADIAN.)
);
#57904=(
NAMED_UNIT(*)
SI_UNIT($,.STERADIAN.)
SOLID_ANGLE_UNIT()
);
#57927=SHAPE_DEFINITION_REPRESENTATION(#57990,#58131);
#57990=PRODUCT_DEFINITION_SHAPE('',$,#58190);
#58131=SHAPE_REPRESENTATION('',(#14651),#57864);
#58167=PRODUCT_DEFINITION_CONTEXT('part definition',#58343,'design');
#58190=PRODUCT_DEFINITION('Carrier plate','Carrier plate',#58248,#58167);
#58248=PRODUCT_DEFINITION_FORMATION('',$,#58367);
#58343=APPLICATION_CONTEXT(
'Core Data for Automotive Mechanical Design Process');
#58344=PRODUCT_CONTEXT('part definition',#58343,'mechanical');
#58367=PRODUCT('Carrier plate','Carrier plate','Carrier plate',(#58344));
#58445=COLOUR_RGB('Light Blue',0.38,0.62,0.78);
#58446=FILL_AREA_STYLE_COLOUR('',#58445);
#58447=FILL_AREA_STYLE('',(#58446));
#58448=SURFACE_STYLE_FILL_AREA(#58447);
#58449=SURFACE_SIDE_STYLE('',(#58448));
#58450=SURFACE_STYLE_USAGE(.BOTH.,#58449);
#58451=PRESENTATION_STYLE_ASSIGNMENT((#58450));
ENDSEC;
END-ISO-10303-21;
